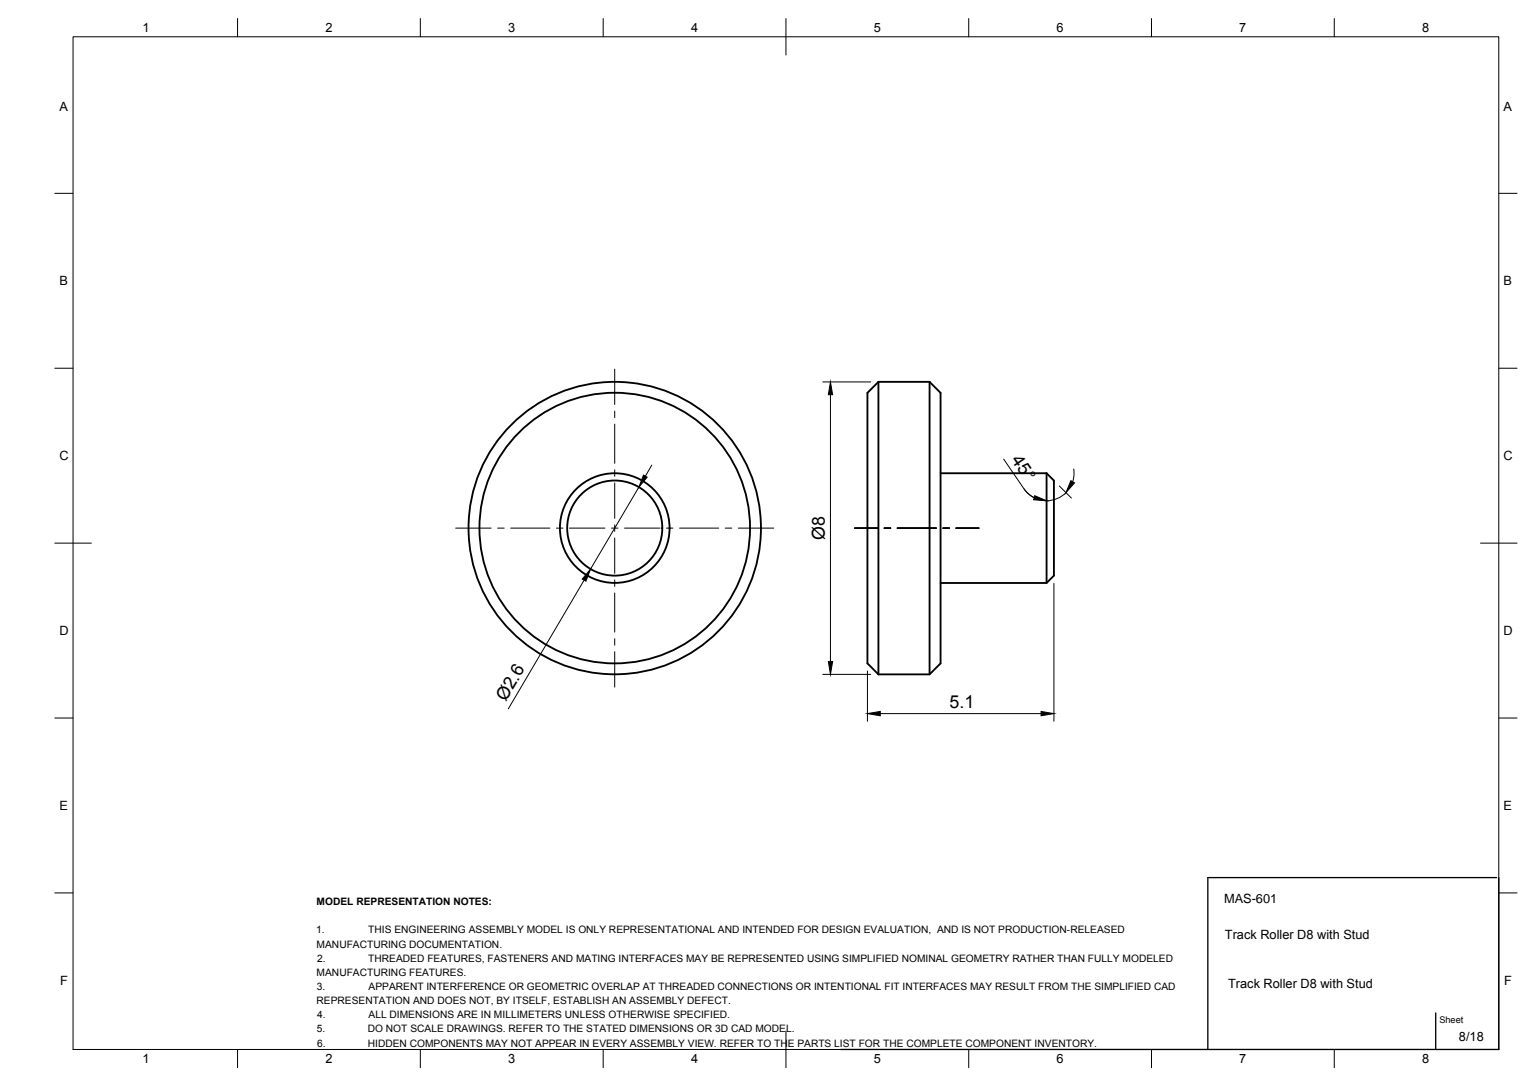
ISO-10303-21;
HEADER;
FILE_DESCRIPTION((''),'2;1');
FILE_NAME('Track Roller D8 with Stud.step','2026-10-06T07:37:42+05:00',(''),(''),'','','');
FILE_SCHEMA (('AUTOMOTIVE_DESIGN { 1 0 10303 214 3 1 1 }'));
ENDSEC;
DATA;
#10=MECHANICAL_DESIGN_GEOMETRIC_PRESENTATION_REPRESENTATION('',(#385),#18757);
#351=SHAPE_REPRESENTATION_RELATIONSHIP('SRR','None',#18869,#368) ;
#368=ADVANCED_BREP_SHAPE_REPRESENTATION('',(#402),#18752) ;
#385=STYLED_ITEM('',(#18963),#402) ;
#402=MANIFOLD_SOLID_BREP('Track Roller D8 with Stud',#9554) ;
#594=CYLINDRICAL_SURFACE('',#10259,4.) ;
#595=CYLINDRICAL_SURFACE('',#10265,1.5) ;
#732=FACE_BOUND('',#1969,.T.) ;
#917=PLANE('',#10255) ;
#918=PLANE('',#10263) ;
#919=PLANE('',#10269) ;
#1364=FACE_OUTER_BOUND('',#1964,.T.) ;
#1365=FACE_OUTER_BOUND('',#1965,.T.) ;
#1366=FACE_OUTER_BOUND('',#1966,.T.) ;
#1367=FACE_OUTER_BOUND('',#1967,.T.) ;
#1368=FACE_OUTER_BOUND('',#1968,.T.) ;
#1369=FACE_OUTER_BOUND('',#1970,.T.) ;
#1370=FACE_OUTER_BOUND('',#1971,.T.) ;
#1371=FACE_OUTER_BOUND('',#1972,.T.) ;
#1964=EDGE_LOOP('',(#7705)) ;
#1965=EDGE_LOOP('',(#7706,#7707,#7708,#7709)) ;
#1966=EDGE_LOOP('',(#7710,#7711,#7712,#7713)) ;
#1967=EDGE_LOOP('',(#7714,#7715,#7716,#7717)) ;
#1968=EDGE_LOOP('',(#7718)) ;
#1969=EDGE_LOOP('',(#7719)) ;
#1970=EDGE_LOOP('',(#7720,#7721,#7722,#7723)) ;
#1971=EDGE_LOOP('',(#7724,#7725,#7726,#7727)) ;
#1972=EDGE_LOOP('',(#7728)) ;
#2666=LINE('',#15277,#3437) ;
#2667=LINE('',#15281,#3438) ;
#2668=LINE('',#15285,#3439) ;
#2669=LINE('',#15292,#3440) ;
#2670=LINE('',#15296,#3441) ;
#3437=VECTOR('',#12172,3.85000000000001) ;
#3438=VECTOR('',#12177,4.) ;
#3439=VECTOR('',#12182,3.85000000000001) ;
#3440=VECTOR('',#12191,1.5) ;
#3441=VECTOR('',#12196,1.40000000000001) ;
#3992=CIRCLE('',#10256,3.70000000000001) ;
#3993=CIRCLE('',#10258,4.) ;
#3994=CIRCLE('',#10260,4.) ;
#3995=CIRCLE('',#10262,3.70000000000001) ;
#3996=CIRCLE('',#10264,1.5) ;
#3997=CIRCLE('',#10266,1.5) ;
#3998=CIRCLE('',#10268,1.3) ;
#4597=VERTEX_POINT('',#15272) ;
#4598=VERTEX_POINT('',#15275) ;
#4599=VERTEX_POINT('',#15279) ;
#4600=VERTEX_POINT('',#15283) ;
#4601=VERTEX_POINT('',#15287) ;
#4602=VERTEX_POINT('',#15290) ;
#4603=VERTEX_POINT('',#15294) ;
#5699=EDGE_CURVE('',#4597,#4597,#3992,.T.) ;
#5700=EDGE_CURVE('',#4598,#4598,#3993,.T.) ;
#5701=EDGE_CURVE('',#4598,#4597,#2666,.T.) ;
#5702=EDGE_CURVE('',#4599,#4599,#3994,.T.) ;
#5703=EDGE_CURVE('',#4599,#4598,#2667,.T.) ;
#5704=EDGE_CURVE('',#4600,#4600,#3995,.T.) ;
#5705=EDGE_CURVE('',#4600,#4599,#2668,.T.) ;
#5706=EDGE_CURVE('',#4601,#4601,#3996,.T.) ;
#5707=EDGE_CURVE('',#4602,#4602,#3997,.T.) ;
#5708=EDGE_CURVE('',#4602,#4601,#2669,.T.) ;
#5709=EDGE_CURVE('',#4603,#4603,#3998,.T.) ;
#5710=EDGE_CURVE('',#4603,#4602,#2670,.T.) ;
#7705=ORIENTED_EDGE('',*,*,#5699,.F.) ;
#7706=ORIENTED_EDGE('',*,*,#5700,.F.) ;
#7707=ORIENTED_EDGE('',*,*,#5701,.T.) ;
#7708=ORIENTED_EDGE('',*,*,#5699,.T.) ;
#7709=ORIENTED_EDGE('',*,*,#5701,.F.) ;
#7710=ORIENTED_EDGE('',*,*,#5702,.F.) ;
#7711=ORIENTED_EDGE('',*,*,#5703,.T.) ;
#7712=ORIENTED_EDGE('',*,*,#5700,.T.) ;
#7713=ORIENTED_EDGE('',*,*,#5703,.F.) ;
#7714=ORIENTED_EDGE('',*,*,#5704,.F.) ;
#7715=ORIENTED_EDGE('',*,*,#5705,.T.) ;
#7716=ORIENTED_EDGE('',*,*,#5702,.T.) ;
#7717=ORIENTED_EDGE('',*,*,#5705,.F.) ;
#7718=ORIENTED_EDGE('',*,*,#5704,.T.) ;
#7719=ORIENTED_EDGE('',*,*,#5706,.F.) ;
#7720=ORIENTED_EDGE('',*,*,#5707,.F.) ;
#7721=ORIENTED_EDGE('',*,*,#5708,.T.) ;
#7722=ORIENTED_EDGE('',*,*,#5706,.T.) ;
#7723=ORIENTED_EDGE('',*,*,#5708,.F.) ;
#7724=ORIENTED_EDGE('',*,*,#5709,.F.) ;
#7725=ORIENTED_EDGE('',*,*,#5710,.T.) ;
#7726=ORIENTED_EDGE('',*,*,#5707,.T.) ;
#7727=ORIENTED_EDGE('',*,*,#5710,.F.) ;
#7728=ORIENTED_EDGE('',*,*,#5709,.T.) ;
#9012=CONICAL_SURFACE('',#10257,3.85000000000001,0.785398163397434) ;
#9013=CONICAL_SURFACE('',#10261,3.85000000000001,0.785398163397448) ;
#9014=CONICAL_SURFACE('',#10267,1.40000000000001,0.785398163397448) ;
#9300=ADVANCED_FACE('',(#1364),#917,.T.) ;
#9301=ADVANCED_FACE('',(#1365),#9012,.T.) ;
#9302=ADVANCED_FACE('',(#1366),#594,.T.) ;
#9303=ADVANCED_FACE('',(#1367),#9013,.T.) ;
#9304=ADVANCED_FACE('',(#1368,#732),#918,.T.) ;
#9305=ADVANCED_FACE('',(#1369),#595,.T.) ;
#9306=ADVANCED_FACE('',(#1370),#9014,.T.) ;
#9307=ADVANCED_FACE('',(#1371),#919,.T.) ;
#9554=CLOSED_SHELL('',(#9300,#9301,#9302,#9303,#9304,#9305,#9306,#9307)) ;
#10254=AXIS2_PLACEMENT_3D('',#15270,#12162,#12163) ;
#10255=AXIS2_PLACEMENT_3D('',#15271,#12164,#12165) ;
#10256=AXIS2_PLACEMENT_3D('',#15273,#12166,#12167) ;
#10257=AXIS2_PLACEMENT_3D('',#15274,#12168,#12169) ;
#10258=AXIS2_PLACEMENT_3D('',#15276,#12170,#12171) ;
#10259=AXIS2_PLACEMENT_3D('',#15278,#12173,#12174) ;
#10260=AXIS2_PLACEMENT_3D('',#15280,#12175,#12176) ;
#10261=AXIS2_PLACEMENT_3D('',#15282,#12178,#12179) ;
#10262=AXIS2_PLACEMENT_3D('',#15284,#12180,#12181) ;
#10263=AXIS2_PLACEMENT_3D('',#15286,#12183,#12184) ;
#10264=AXIS2_PLACEMENT_3D('',#15288,#12185,#12186) ;
#10265=AXIS2_PLACEMENT_3D('',#15289,#12187,#12188) ;
#10266=AXIS2_PLACEMENT_3D('',#15291,#12189,#12190) ;
#10267=AXIS2_PLACEMENT_3D('',#15293,#12192,#12193) ;
#10268=AXIS2_PLACEMENT_3D('',#15295,#12194,#12195) ;
#10269=AXIS2_PLACEMENT_3D('',#15297,#12197,#12198) ;
#12162=DIRECTION('axis',(0.,0.,1.)) ;
#12163=DIRECTION('refdir',(1.,0.,0.)) ;
#12164=DIRECTION('center_axis',(0.,1.,0.)) ;
#12165=DIRECTION('ref_axis',(0.,0.,1.)) ;
#12166=DIRECTION('center_axis',(0.,-1.,0.)) ;
#12167=DIRECTION('ref_axis',(1.,0.,0.)) ;
#12168=DIRECTION('center_axis',(0.,-1.,0.)) ;
#12169=DIRECTION('ref_axis',(1.,0.,0.)) ;
#12170=DIRECTION('center_axis',(0.,-1.,0.)) ;
#12171=DIRECTION('ref_axis',(1.,0.,0.)) ;
#12172=DIRECTION('',(0.707106781186537,0.707106781186558,8.6595605623548E-17)) ;
#12173=DIRECTION('center_axis',(0.,-1.,0.)) ;
#12174=DIRECTION('ref_axis',(1.,0.,0.)) ;
#12175=DIRECTION('center_axis',(0.,-1.,0.)) ;
#12176=DIRECTION('ref_axis',(1.,0.,0.)) ;
#12177=DIRECTION('',(0.,1.,0.)) ;
#12178=DIRECTION('center_axis',(0.,1.,0.)) ;
#12179=DIRECTION('ref_axis',(1.,0.,0.)) ;
#12180=DIRECTION('center_axis',(0.,-1.,0.)) ;
#12181=DIRECTION('ref_axis',(1.,0.,0.)) ;
#12182=DIRECTION('',(-0.707106781186547,0.707106781186547,-8.65956056235493E-17)) ;
#12183=DIRECTION('center_axis',(0.,-1.,0.)) ;
#12184=DIRECTION('ref_axis',(0.,0.,-1.)) ;
#12185=DIRECTION('center_axis',(0.,-1.,0.)) ;
#12186=DIRECTION('ref_axis',(1.,0.,0.)) ;
#12187=DIRECTION('center_axis',(0.,-1.,0.)) ;
#12188=DIRECTION('ref_axis',(1.,0.,0.)) ;
#12189=DIRECTION('center_axis',(0.,-1.,0.)) ;
#12190=DIRECTION('ref_axis',(1.,0.,0.)) ;
#12191=DIRECTION('',(0.,1.,0.)) ;
#12192=DIRECTION('center_axis',(0.,1.,0.)) ;
#12193=DIRECTION('ref_axis',(1.,0.,0.)) ;
#12194=DIRECTION('center_axis',(0.,-1.,0.)) ;
#12195=DIRECTION('ref_axis',(1.,0.,0.)) ;
#12196=DIRECTION('',(-0.707106781186548,0.707106781186548,-8.65956056235493E-17)) ;
#12197=DIRECTION('center_axis',(0.,-1.,0.)) ;
#12198=DIRECTION('ref_axis',(0.,0.,-1.)) ;
#15270=CARTESIAN_POINT('',(0.,0.,0.)) ;
#15271=CARTESIAN_POINT('Origin',(-68.9949895469777,49.9,44.4)) ;
#15272=CARTESIAN_POINT('',(-76.3949895469778,49.9,44.4)) ;
#15273=CARTESIAN_POINT('Origin',(-72.6949895469778,49.9,44.4)) ;
#15274=CARTESIAN_POINT('Origin',(-72.6949895469778,49.75,44.4)) ;
#15275=CARTESIAN_POINT('',(-76.6949895469778,49.6,44.4)) ;
#15276=CARTESIAN_POINT('Origin',(-72.6949895469778,49.6,44.4)) ;
#15277=CARTESIAN_POINT('',(-76.5449895469778,49.75,44.4)) ;
#15278=CARTESIAN_POINT('Origin',(-72.6949895469778,48.9,44.4)) ;
#15279=CARTESIAN_POINT('',(-76.6949895469778,48.2,44.4)) ;
#15280=CARTESIAN_POINT('Origin',(-72.6949895469778,48.2,44.4)) ;
#15281=CARTESIAN_POINT('',(-76.6949895469778,48.9,44.4)) ;
#15282=CARTESIAN_POINT('Origin',(-72.6949895469778,48.05,44.4)) ;
#15283=CARTESIAN_POINT('',(-76.3949895469778,47.9,44.4)) ;
#15284=CARTESIAN_POINT('Origin',(-72.6949895469778,47.9,44.4)) ;
#15285=CARTESIAN_POINT('',(-76.5449895469778,48.05,44.4)) ;
#15286=CARTESIAN_POINT('Origin',(-71.1949895469778,47.9,44.4)) ;
#15287=CARTESIAN_POINT('',(-74.1949895469778,47.9,44.4)) ;
#15288=CARTESIAN_POINT('Origin',(-72.6949895469778,47.9,44.4)) ;
#15289=CARTESIAN_POINT('Origin',(-72.6949895469778,46.45,44.4)) ;
#15290=CARTESIAN_POINT('',(-74.1949895469778,45.,44.4)) ;
#15291=CARTESIAN_POINT('Origin',(-72.6949895469778,45.,44.4)) ;
#15292=CARTESIAN_POINT('',(-74.1949895469778,46.45,44.4)) ;
#15293=CARTESIAN_POINT('Origin',(-72.6949895469778,44.9,44.4)) ;
#15294=CARTESIAN_POINT('',(-73.9949895469777,44.8,44.4)) ;
#15295=CARTESIAN_POINT('Origin',(-72.6949895469778,44.8,44.4)) ;
#15296=CARTESIAN_POINT('',(-74.0949895469778,44.9,44.4)) ;
#15297=CARTESIAN_POINT('Origin',(-72.6949895469778,44.8,44.4)) ;
#18733=UNCERTAINTY_MEASURE_WITH_UNIT(LENGTH_MEASURE(0.01),#18758,
'DISTANCE_ACCURACY_VALUE',
'Maximum model space distance between geometric entities at asserted c
onnectivities') ;
#18738=UNCERTAINTY_MEASURE_WITH_UNIT(LENGTH_MEASURE(0.01),#18758,
'DISTANCE_ACCURACY_VALUE',
'Maximum model space distance between geometric entities at asserted c
onnectivities') ;
#18752=(
GEOMETRIC_REPRESENTATION_CONTEXT(3)
GLOBAL_UNCERTAINTY_ASSIGNED_CONTEXT((#18733))
GLOBAL_UNIT_ASSIGNED_CONTEXT((#18758,#18760,#18761))
REPRESENTATION_CONTEXT('','3D')
) ;
#18757=(
GEOMETRIC_REPRESENTATION_CONTEXT(3)
GLOBAL_UNCERTAINTY_ASSIGNED_CONTEXT((#18738))
GLOBAL_UNIT_ASSIGNED_CONTEXT((#18758,#18760,#18761))
REPRESENTATION_CONTEXT('','3D')
) ;
#18758=(
LENGTH_UNIT()
NAMED_UNIT(*)
SI_UNIT(.MILLI.,.METRE.)
) ;
#18760=(
NAMED_UNIT(*)
PLANE_ANGLE_UNIT()
SI_UNIT($,.RADIAN.)
) ;
#18761=(
NAMED_UNIT(*)
SI_UNIT($,.STERADIAN.)
SOLID_ANGLE_UNIT()
) ;
#18775=SHAPE_DEFINITION_REPRESENTATION(#18793,#18869) ;
#18793=PRODUCT_DEFINITION_SHAPE('',$,#18888) ;
#18869=SHAPE_REPRESENTATION('',(#10254),#18752) ;
#18874=PRODUCT_DEFINITION_CONTEXT('part definition',#18930,'design') ;
#18888=PRODUCT_DEFINITION('Track Roller D8 with Stud',
'Track Roller D8 with Stud',#18906,#18874) ;
#18906=PRODUCT_DEFINITION_FORMATION('',$,#18945) ;
#18930=APPLICATION_CONTEXT(
'Core Data for Automotive Mechanical Design Process') ;
#18931=PRODUCT_CONTEXT('part definition',#18930,'mechanical') ;
#18945=PRODUCT('Track Roller D8 with Stud','Track Roller D8 with Stud',$,
(#18931)) ;
#18963=PRESENTATION_STYLE_ASSIGNMENT((#18981)) ;
#18981=SURFACE_STYLE_USAGE(.BOTH.,#18999) ;
#18999=SURFACE_SIDE_STYLE('',(#19017)) ;
#19017=SURFACE_STYLE_FILL_AREA(#19035) ;
#19035=FILL_AREA_STYLE(
'MAS-253 Metallic Sheet - Track Roller D8 with Stud',(#19053)) ;
#19053=FILL_AREA_STYLE_COLOUR(
'MAS-253 Metallic Sheet - Track Roller D8 with Stud',#19071) ;
#19071=COLOUR_RGB('MAS-253 Metallic Sheet - Track Roller D8 with Stud', 0.66274510, 0.83137255, 0.94901961) ;
ENDSEC;
END-ISO-10303-21;
